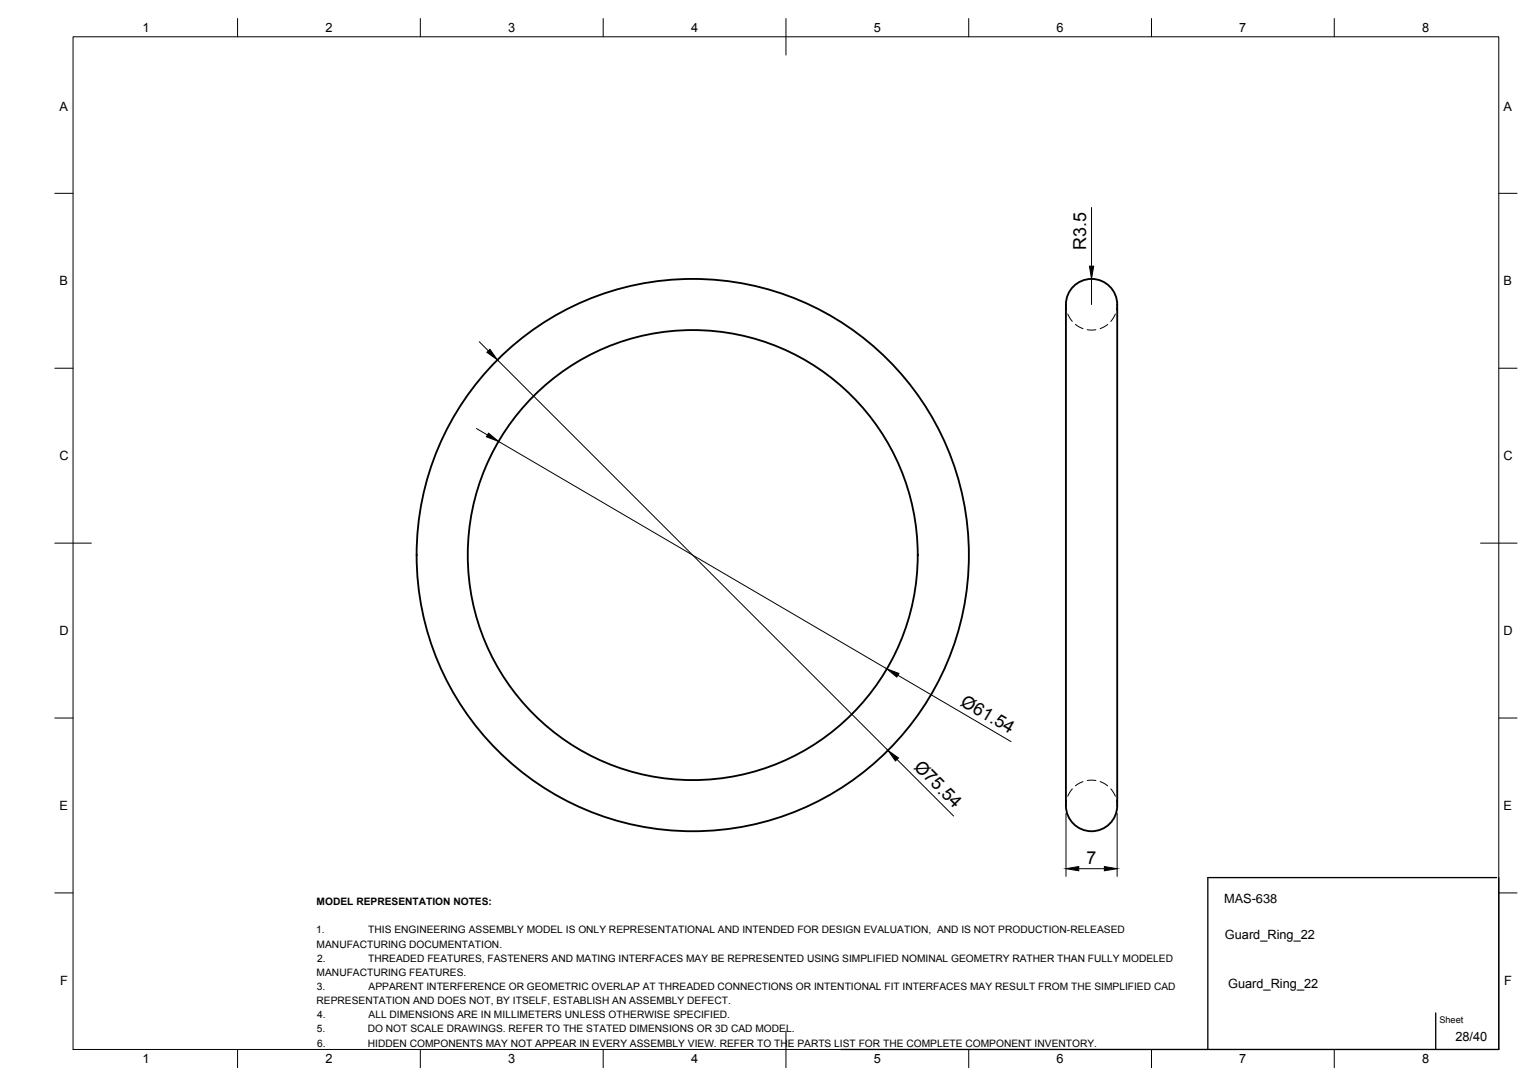
ISO-10303-21;
HEADER;
FILE_DESCRIPTION((''),'2;1');
FILE_NAME('Guard_Ring_22.step','2026-10-09T12:00:21-07:00',(''),(''),'','','');
FILE_SCHEMA (('AUTOMOTIVE_DESIGN { 1 0 10303 214 3 1 1 }'));
ENDSEC;
DATA;
#10=MECHANICAL_DESIGN_GEOMETRIC_PRESENTATION_REPRESENTATION('',(#427),#10334);
#355=SHAPE_REPRESENTATION_RELATIONSHIP('SRR','None',#10471,#387) ;
#387=ADVANCED_BREP_SHAPE_REPRESENTATION('',(#459),#10323) ;
#427=STYLED_ITEM('',(#10632),#459) ;
#459=MANIFOLD_SOLID_BREP('Body1',#3581) ;
#880=FACE_OUTER_BOUND('',#1080,.T.) ;
#1080=EDGE_LOOP('',(#2433,#2434,#2435,#2436)) ;
#1318=CIRCLE('',#4059,0.349999999999999) ;
#1319=CIRCLE('',#4060,3.07681446136678) ;
#1534=VERTEX_POINT('',#5758) ;
#1873=EDGE_CURVE('',#1534,#1534,#1318,.T.) ;
#1874=EDGE_CURVE('',#1534,#1534,#1319,.T.) ;
#2433=ORIENTED_EDGE('',*,*,#1873,.F.) ;
#2434=ORIENTED_EDGE('',*,*,#1874,.T.) ;
#2435=ORIENTED_EDGE('',*,*,#1873,.T.) ;
#2436=ORIENTED_EDGE('',*,*,#1874,.F.) ;
#3326=TOROIDAL_SURFACE('',#4058,3.42681446136678,0.349999999999999) ;
#3388=ADVANCED_FACE('',(#880),#3326,.T.) ;
#3581=CLOSED_SHELL('',(#3388)) ;
#4057=AXIS2_PLACEMENT_3D('',#5756,#4675,#4676) ;
#4058=AXIS2_PLACEMENT_3D('',#5757,#4677,#4678) ;
#4059=AXIS2_PLACEMENT_3D('',#5759,#4679,#4680) ;
#4060=AXIS2_PLACEMENT_3D('',#5760,#4681,#4682) ;
#4675=DIRECTION('axis',(0.,0.,1.)) ;
#4676=DIRECTION('refdir',(1.,0.,0.)) ;
#4677=DIRECTION('center_axis',(-6.42891162084177E-17,-1.,-1.01883556321148E-16)) ;
#4678=DIRECTION('ref_axis',(1.,0.,0.)) ;
#4679=DIRECTION('center_axis',(0.,1.01883556321148E-16,-1.)) ;
#4680=DIRECTION('ref_axis',(-1.,0.,0.)) ;
#4681=DIRECTION('center_axis',(6.42891162084177E-17,1.,1.01883556321148E-16)) ;
#4682=DIRECTION('ref_axis',(1.,-6.42891162084177E-17,-6.55000379205715E-33)) ;
#5756=CARTESIAN_POINT('',(0.,0.,0.)) ;
#5757=CARTESIAN_POINT('Origin',(23.47768801576,62.6831179463143,68.2224337400009)) ;
#5758=CARTESIAN_POINT('',(20.4008735543932,62.6831179463143,68.2224337400009)) ;
#5759=CARTESIAN_POINT('Origin',(20.0508735543932,62.6831179463143,68.2224337400009)) ;
#5760=CARTESIAN_POINT('Origin',(23.47768801576,62.6831179463143,68.2224337400009)) ;
#10286=UNCERTAINTY_MEASURE_WITH_UNIT(LENGTH_MEASURE(0.001),#10335,
'DISTANCE_ACCURACY_VALUE',
'Maximum model space distance between geometric entities at asserted c
onnectivities') ;
#10297=UNCERTAINTY_MEASURE_WITH_UNIT(LENGTH_MEASURE(0.001),#10335,
'DISTANCE_ACCURACY_VALUE',
'Maximum model space distance between geometric entities at asserted c
onnectivities') ;
#10323=(
GEOMETRIC_REPRESENTATION_CONTEXT(3)
GLOBAL_UNCERTAINTY_ASSIGNED_CONTEXT((#10286))
GLOBAL_UNIT_ASSIGNED_CONTEXT((#10335,#10337,#10338))
REPRESENTATION_CONTEXT('','3D')
) ;
#10334=(
GEOMETRIC_REPRESENTATION_CONTEXT(3)
GLOBAL_UNCERTAINTY_ASSIGNED_CONTEXT((#10297))
GLOBAL_UNIT_ASSIGNED_CONTEXT((#10335,#10337,#10338))
REPRESENTATION_CONTEXT('','3D')
) ;
#10335=(
LENGTH_UNIT()
NAMED_UNIT(*)
SI_UNIT(.CENTI.,.METRE.)
) ;
#10337=(
NAMED_UNIT(*)
PLANE_ANGLE_UNIT()
SI_UNIT($,.RADIAN.)
) ;
#10338=(
NAMED_UNIT(*)
SI_UNIT($,.STERADIAN.)
SOLID_ANGLE_UNIT()
) ;
#10364=SHAPE_DEFINITION_REPRESENTATION(#10400,#10471) ;
#10400=PRODUCT_DEFINITION_SHAPE('',$,#10508) ;
#10471=SHAPE_REPRESENTATION('',(#4057),#10323) ;
#10482=PRODUCT_DEFINITION_CONTEXT('part definition',#10592,'design') ;
#10508=PRODUCT_DEFINITION('Guard_Ring_22','Guard_Ring_22',#10544,#10482) ;
#10544=PRODUCT_DEFINITION_FORMATION('',$,#10619) ;
#10592=APPLICATION_CONTEXT(
'Core Data for Automotive Mechanical Design Process') ;
#10593=PRODUCT_CONTEXT('part definition',#10592,'mechanical') ;
#10619=PRODUCT('Guard_Ring_22','Guard_Ring_22',$,(#10593)) ;
#10632=PRESENTATION_STYLE_ASSIGNMENT((#10636)) ;
#10636=SURFACE_STYLE_USAGE(.BOTH.,#10640) ;
#10640=SURFACE_SIDE_STYLE('',(#10644)) ;
#10644=SURFACE_STYLE_FILL_AREA(#10648) ;
#10648=FILL_AREA_STYLE('Opaque(202,209,238)',(#10652)) ;
#10652=FILL_AREA_STYLE_COLOUR('Opaque(202,209,238)',#10656) ;
#10656=COLOUR_RGB('Opaque(202,209,238)', 0.40784314, 0.44705882, 0.49803922) ;
ENDSEC;
END-ISO-10303-21;
